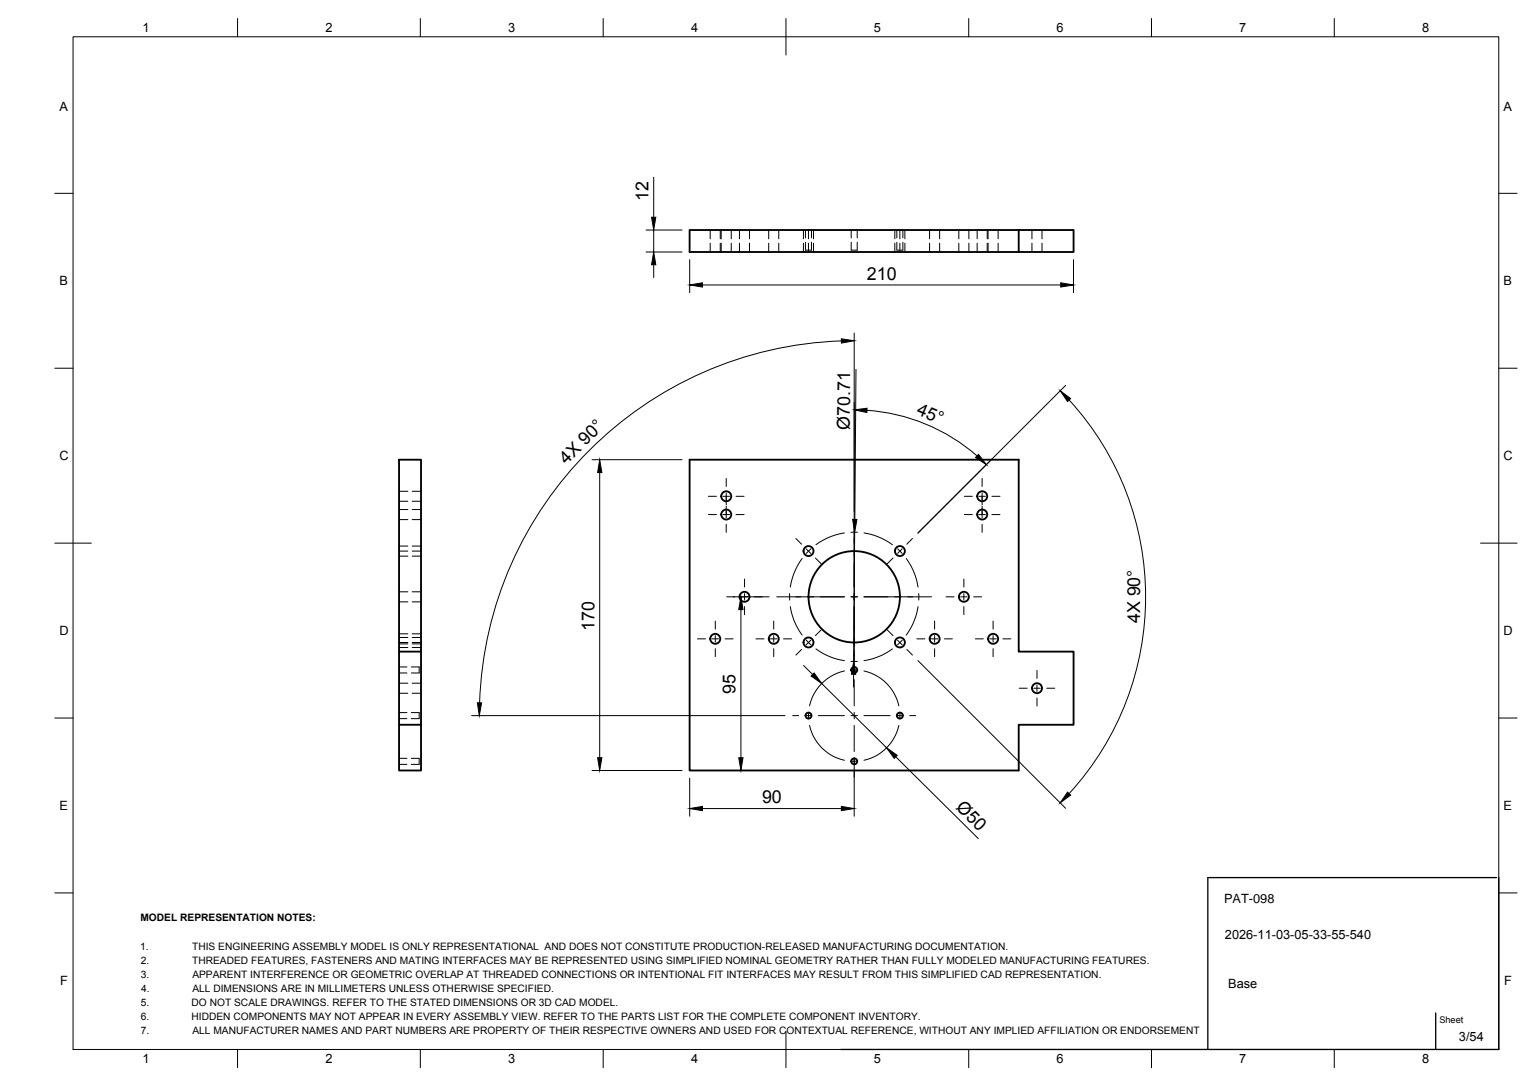
ISO-10303-21;
HEADER;
/* Generated by software containing ST-Developer
 * from STEP Tools, Inc. (www.steptools.com) 
 */

FILE_DESCRIPTION(
/* description */ ('Spring compression tester'),
/* implementation_level */ '2;1');

FILE_NAME(
/* name */ 'Base.step',
/* time_stamp */ '2026-10-28T03:24:11-07:00',
/* author */ (''),
/* organization */ (''),
/* preprocessor_version */ 'ST-DEVELOPER v20.2',
/* originating_system */ 'Autodesk Translation Framework v15.17.0.0',
/* authorisation */ '');

FILE_SCHEMA (('AUTOMOTIVE_DESIGN { 1 0 10303 214 3 1 1 }'));
ENDSEC;

DATA;
#10=MECHANICAL_DESIGN_GEOMETRIC_PRESENTATION_REPRESENTATION('',(#1104),#43521);
#984=SHAPE_REPRESENTATION_RELATIONSHIP('SRR','None',#43796,#1044);
#1044=ADVANCED_BREP_SHAPE_REPRESENTATION('',(#1179),#43456);
#1104=STYLED_ITEM('',(#44181),#1179);
#1179=MANIFOLD_SOLID_BREP('Body1',#18541);
#1247=FACE_BOUND('',#3250,.T.);
#1248=FACE_BOUND('',#3251,.T.);
#1249=FACE_BOUND('',#3252,.T.);
#1250=FACE_BOUND('',#3253,.T.);
#1251=FACE_BOUND('',#3254,.T.);
#1252=FACE_BOUND('',#3255,.T.);
#1253=FACE_BOUND('',#3256,.T.);
#1254=FACE_BOUND('',#3257,.T.);
#1255=FACE_BOUND('',#3258,.T.);
#1256=FACE_BOUND('',#3259,.T.);
#1257=FACE_BOUND('',#3260,.T.);
#1258=FACE_BOUND('',#3261,.T.);
#1259=FACE_BOUND('',#3262,.T.);
#1260=FACE_BOUND('',#3263,.T.);
#1261=FACE_BOUND('',#3264,.T.);
#1262=FACE_BOUND('',#3265,.T.);
#1263=FACE_BOUND('',#3266,.T.);
#1264=FACE_BOUND('',#3267,.T.);
#1265=FACE_BOUND('',#3268,.T.);
#1266=FACE_BOUND('',#3269,.T.);
#1267=FACE_BOUND('',#3271,.T.);
#1268=FACE_BOUND('',#3272,.T.);
#1269=FACE_BOUND('',#3273,.T.);
#1270=FACE_BOUND('',#3274,.T.);
#1271=FACE_BOUND('',#3275,.T.);
#1272=FACE_BOUND('',#3276,.T.);
#1273=FACE_BOUND('',#3277,.T.);
#1274=FACE_BOUND('',#3278,.T.);
#1275=FACE_BOUND('',#3279,.T.);
#1276=FACE_BOUND('',#3280,.T.);
#1277=FACE_BOUND('',#3281,.T.);
#1278=FACE_BOUND('',#3282,.T.);
#1279=FACE_BOUND('',#3283,.T.);
#1280=FACE_BOUND('',#3284,.T.);
#1281=FACE_BOUND('',#3285,.T.);
#1282=FACE_BOUND('',#3286,.T.);
#1589=PLANE('',#19290);
#1590=PLANE('',#19291);
#1591=PLANE('',#19292);
#1592=PLANE('',#19293);
#1593=PLANE('',#19294);
#1594=PLANE('',#19298);
#1595=PLANE('',#19302);
#1596=PLANE('',#19306);
#1597=PLANE('',#19310);
#1598=PLANE('',#19356);
#1599=PLANE('',#19357);
#1600=PLANE('',#19358);
#1601=PLANE('',#19359);
#1602=PLANE('',#19360);
#2170=FACE_OUTER_BOUND('',#3217,.T.);
#2171=FACE_OUTER_BOUND('',#3218,.T.);
#2172=FACE_OUTER_BOUND('',#3219,.T.);
#2173=FACE_OUTER_BOUND('',#3220,.T.);
#2174=FACE_OUTER_BOUND('',#3221,.T.);
#2175=FACE_OUTER_BOUND('',#3222,.T.);
#2176=FACE_OUTER_BOUND('',#3223,.T.);
#2177=FACE_OUTER_BOUND('',#3224,.T.);
#2178=FACE_OUTER_BOUND('',#3225,.T.);
#2179=FACE_OUTER_BOUND('',#3226,.T.);
#2180=FACE_OUTER_BOUND('',#3227,.T.);
#2181=FACE_OUTER_BOUND('',#3228,.T.);
#2182=FACE_OUTER_BOUND('',#3229,.T.);
#2183=FACE_OUTER_BOUND('',#3230,.T.);
#2184=FACE_OUTER_BOUND('',#3231,.T.);
#2185=FACE_OUTER_BOUND('',#3232,.T.);
#2186=FACE_OUTER_BOUND('',#3233,.T.);
#2187=FACE_OUTER_BOUND('',#3234,.T.);
#2188=FACE_OUTER_BOUND('',#3235,.T.);
#2189=FACE_OUTER_BOUND('',#3236,.T.);
#2190=FACE_OUTER_BOUND('',#3237,.T.);
#2191=FACE_OUTER_BOUND('',#3238,.T.);
#2192=FACE_OUTER_BOUND('',#3239,.T.);
#2193=FACE_OUTER_BOUND('',#3240,.T.);
#2194=FACE_OUTER_BOUND('',#3241,.T.);
#2195=FACE_OUTER_BOUND('',#3242,.T.);
#2196=FACE_OUTER_BOUND('',#3243,.T.);
#2197=FACE_OUTER_BOUND('',#3244,.T.);
#2198=FACE_OUTER_BOUND('',#3245,.T.);
#2199=FACE_OUTER_BOUND('',#3246,.T.);
#2200=FACE_OUTER_BOUND('',#3247,.T.);
#2201=FACE_OUTER_BOUND('',#3248,.T.);
#2202=FACE_OUTER_BOUND('',#3249,.T.);
#2203=FACE_OUTER_BOUND('',#3270,.T.);
#3217=EDGE_LOOP('',(#12217,#12218,#12219,#12220));
#3218=EDGE_LOOP('',(#12221,#12222,#12223,#12224));
#3219=EDGE_LOOP('',(#12225,#12226,#12227,#12228));
#3220=EDGE_LOOP('',(#12229,#12230,#12231,#12232));
#3221=EDGE_LOOP('',(#12233,#12234,#12235,#12236));
#3222=EDGE_LOOP('',(#12237,#12238,#12239,#12240));
#3223=EDGE_LOOP('',(#12241,#12242,#12243,#12244));
#3224=EDGE_LOOP('',(#12245));
#3225=EDGE_LOOP('',(#12246,#12247,#12248,#12249));
#3226=EDGE_LOOP('',(#12250));
#3227=EDGE_LOOP('',(#12251,#12252,#12253,#12254));
#3228=EDGE_LOOP('',(#12255));
#3229=EDGE_LOOP('',(#12256,#12257,#12258,#12259));
#3230=EDGE_LOOP('',(#12260));
#3231=EDGE_LOOP('',(#12261,#12262,#12263,#12264));
#3232=EDGE_LOOP('',(#12265,#12266,#12267,#12268));
#3233=EDGE_LOOP('',(#12269,#12270,#12271,#12272));
#3234=EDGE_LOOP('',(#12273,#12274,#12275,#12276));
#3235=EDGE_LOOP('',(#12277,#12278,#12279,#12280));
#3236=EDGE_LOOP('',(#12281,#12282,#12283,#12284));
#3237=EDGE_LOOP('',(#12285,#12286,#12287,#12288));
#3238=EDGE_LOOP('',(#12289,#12290,#12291,#12292));
#3239=EDGE_LOOP('',(#12293,#12294,#12295,#12296));
#3240=EDGE_LOOP('',(#12297,#12298,#12299,#12300));
#3241=EDGE_LOOP('',(#12301,#12302,#12303,#12304));
#3242=EDGE_LOOP('',(#12305,#12306,#12307,#12308));
#3243=EDGE_LOOP('',(#12309,#12310,#12311,#12312));
#3244=EDGE_LOOP('',(#12313,#12314,#12315,#12316));
#3245=EDGE_LOOP('',(#12317,#12318,#12319,#12320));
#3246=EDGE_LOOP('',(#12321,#12322,#12323,#12324));
#3247=EDGE_LOOP('',(#12325,#12326,#12327,#12328));
#3248=EDGE_LOOP('',(#12329,#12330,#12331,#12332));
#3249=EDGE_LOOP('',(#12333,#12334,#12335,#12336,#12337,#12338,#12339,#12340));
#3250=EDGE_LOOP('',(#12341));
#3251=EDGE_LOOP('',(#12342));
#3252=EDGE_LOOP('',(#12343));
#3253=EDGE_LOOP('',(#12344));
#3254=EDGE_LOOP('',(#12345));
#3255=EDGE_LOOP('',(#12346));
#3256=EDGE_LOOP('',(#12347));
#3257=EDGE_LOOP('',(#12348));
#3258=EDGE_LOOP('',(#12349));
#3259=EDGE_LOOP('',(#12350));
#3260=EDGE_LOOP('',(#12351));
#3261=EDGE_LOOP('',(#12352));
#3262=EDGE_LOOP('',(#12353));
#3263=EDGE_LOOP('',(#12354));
#3264=EDGE_LOOP('',(#12355));
#3265=EDGE_LOOP('',(#12356));
#3266=EDGE_LOOP('',(#12357));
#3267=EDGE_LOOP('',(#12358));
#3268=EDGE_LOOP('',(#12359));
#3269=EDGE_LOOP('',(#12360));
#3270=EDGE_LOOP('',(#12361,#12362,#12363,#12364,#12365,#12366,#12367,#12368));
#3271=EDGE_LOOP('',(#12369));
#3272=EDGE_LOOP('',(#12370));
#3273=EDGE_LOOP('',(#12371));
#3274=EDGE_LOOP('',(#12372));
#3275=EDGE_LOOP('',(#12373));
#3276=EDGE_LOOP('',(#12374));
#3277=EDGE_LOOP('',(#12375));
#3278=EDGE_LOOP('',(#12376));
#3279=EDGE_LOOP('',(#12377));
#3280=EDGE_LOOP('',(#12378));
#3281=EDGE_LOOP('',(#12379));
#3282=EDGE_LOOP('',(#12380));
#3283=EDGE_LOOP('',(#12381));
#3284=EDGE_LOOP('',(#12382));
#3285=EDGE_LOOP('',(#12383));
#3286=EDGE_LOOP('',(#12384));
#4606=LINE('',#26459,#6038);
#4607=LINE('',#26464,#6039);
#4608=LINE('',#26466,#6040);
#4609=LINE('',#26468,#6041);
#4610=LINE('',#26469,#6042);
#4611=LINE('',#26473,#6043);
#4612=LINE('',#26474,#6044);
#4613=LINE('',#26475,#6045);
#4614=LINE('',#26479,#6046);
#4615=LINE('',#26480,#6047);
#4616=LINE('',#26481,#6048);
#4617=LINE('',#26484,#6049);
#4618=LINE('',#26486,#6050);
#4619=LINE('',#26487,#6051);
#4620=LINE('',#26490,#6052);
#4621=LINE('',#26492,#6053);
#4622=LINE('',#26493,#6054);
#4623=LINE('',#26498,#6055);
#4624=LINE('',#26505,#6056);
#4625=LINE('',#26512,#6057);
#4626=LINE('',#26519,#6058);
#4627=LINE('',#26526,#6059);
#4628=LINE('',#26532,#6060);
#4629=LINE('',#26538,#6061);
#4630=LINE('',#26544,#6062);
#4631=LINE('',#26550,#6063);
#4632=LINE('',#26556,#6064);
#4633=LINE('',#26562,#6065);
#4634=LINE('',#26568,#6066);
#4635=LINE('',#26574,#6067);
#4636=LINE('',#26580,#6068);
#4637=LINE('',#26586,#6069);
#4638=LINE('',#26592,#6070);
#4639=LINE('',#26598,#6071);
#4640=LINE('',#26604,#6072);
#4641=LINE('',#26610,#6073);
#4642=LINE('',#26614,#6074);
#4643=LINE('',#26616,#6075);
#4644=LINE('',#26617,#6076);
#4645=LINE('',#26620,#6077);
#4646=LINE('',#26622,#6078);
#4647=LINE('',#26623,#6079);
#4648=LINE('',#26625,#6080);
#4649=LINE('',#26626,#6081);
#6038=VECTOR('',#21206,0.275);
#6039=VECTOR('',#21211,1.);
#6040=VECTOR('',#21212,1.);
#6041=VECTOR('',#21213,1.);
#6042=VECTOR('',#21214,1.);
#6043=VECTOR('',#21217,1.);
#6044=VECTOR('',#21218,1.);
#6045=VECTOR('',#21219,1.);
#6046=VECTOR('',#21222,1.);
#6047=VECTOR('',#21223,1.);
#6048=VECTOR('',#21224,1.);
#6049=VECTOR('',#21227,1.);
#6050=VECTOR('',#21228,1.);
#6051=VECTOR('',#21229,1.);
#6052=VECTOR('',#21232,1.);
#6053=VECTOR('',#21233,1.);
#6054=VECTOR('',#21234,1.);
#6055=VECTOR('',#21239,0.165);
#6056=VECTOR('',#21248,0.165);
#6057=VECTOR('',#21257,0.165);
#6058=VECTOR('',#21266,0.165);
#6059=VECTOR('',#21275,0.275);
#6060=VECTOR('',#21282,0.275);
#6061=VECTOR('',#21289,0.275);
#6062=VECTOR('',#21296,0.275);
#6063=VECTOR('',#21303,0.275);
#6064=VECTOR('',#21310,0.275);
#6065=VECTOR('',#21317,2.5);
#6066=VECTOR('',#21324,0.275);
#6067=VECTOR('',#21331,0.275);
#6068=VECTOR('',#21338,0.275);
#6069=VECTOR('',#21345,0.275);
#6070=VECTOR('',#21352,0.275);
#6071=VECTOR('',#21359,0.275);
#6072=VECTOR('',#21366,0.275);
#6073=VECTOR('',#21373,0.275);
#6074=VECTOR('',#21378,1.);
#6075=VECTOR('',#21379,1.);
#6076=VECTOR('',#21380,1.);
#6077=VECTOR('',#21383,1.);
#6078=VECTOR('',#21384,1.);
#6079=VECTOR('',#21385,1.);
#6080=VECTOR('',#21388,1.);
#6081=VECTOR('',#21389,1.);
#7470=CIRCLE('',#19288,0.275);
#7471=CIRCLE('',#19289,0.275);
#7472=CIRCLE('',#19296,0.165);
#7473=CIRCLE('',#19297,0.165);
#7474=CIRCLE('',#19300,0.165);
#7475=CIRCLE('',#19301,0.165);
#7476=CIRCLE('',#19304,0.165);
#7477=CIRCLE('',#19305,0.165);
#7478=CIRCLE('',#19308,0.165);
#7479=CIRCLE('',#19309,0.165);
#7480=CIRCLE('',#19312,0.275);
#7481=CIRCLE('',#19313,0.275);
#7482=CIRCLE('',#19315,0.275);
#7483=CIRCLE('',#19316,0.275);
#7484=CIRCLE('',#19318,0.275);
#7485=CIRCLE('',#19319,0.275);
#7486=CIRCLE('',#19321,0.275);
#7487=CIRCLE('',#19322,0.275);
#7488=CIRCLE('',#19324,0.275);
#7489=CIRCLE('',#19325,0.275);
#7490=CIRCLE('',#19327,0.275);
#7491=CIRCLE('',#19328,0.275);
#7492=CIRCLE('',#19330,2.5);
#7493=CIRCLE('',#19331,2.5);
#7494=CIRCLE('',#19333,0.275);
#7495=CIRCLE('',#19334,0.275);
#7496=CIRCLE('',#19336,0.275);
#7497=CIRCLE('',#19337,0.275);
#7498=CIRCLE('',#19339,0.275);
#7499=CIRCLE('',#19340,0.275);
#7500=CIRCLE('',#19342,0.275);
#7501=CIRCLE('',#19343,0.275);
#7502=CIRCLE('',#19345,0.275);
#7503=CIRCLE('',#19346,0.275);
#7504=CIRCLE('',#19348,0.275);
#7505=CIRCLE('',#19349,0.275);
#7506=CIRCLE('',#19351,0.275);
#7507=CIRCLE('',#19352,0.275);
#7508=CIRCLE('',#19354,0.275);
#7509=CIRCLE('',#19355,0.275);
#8136=VERTEX_POINT('',#26456);
#8137=VERTEX_POINT('',#26458);
#8138=VERTEX_POINT('',#26462);
#8139=VERTEX_POINT('',#26463);
#8140=VERTEX_POINT('',#26465);
#8141=VERTEX_POINT('',#26467);
#8142=VERTEX_POINT('',#26471);
#8143=VERTEX_POINT('',#26472);
#8144=VERTEX_POINT('',#26477);
#8145=VERTEX_POINT('',#26478);
#8146=VERTEX_POINT('',#26483);
#8147=VERTEX_POINT('',#26485);
#8148=VERTEX_POINT('',#26489);
#8149=VERTEX_POINT('',#26491);
#8150=VERTEX_POINT('',#26495);
#8151=VERTEX_POINT('',#26497);
#8152=VERTEX_POINT('',#26502);
#8153=VERTEX_POINT('',#26504);
#8154=VERTEX_POINT('',#26509);
#8155=VERTEX_POINT('',#26511);
#8156=VERTEX_POINT('',#26516);
#8157=VERTEX_POINT('',#26518);
#8158=VERTEX_POINT('',#26523);
#8159=VERTEX_POINT('',#26525);
#8160=VERTEX_POINT('',#26529);
#8161=VERTEX_POINT('',#26531);
#8162=VERTEX_POINT('',#26535);
#8163=VERTEX_POINT('',#26537);
#8164=VERTEX_POINT('',#26541);
#8165=VERTEX_POINT('',#26543);
#8166=VERTEX_POINT('',#26547);
#8167=VERTEX_POINT('',#26549);
#8168=VERTEX_POINT('',#26553);
#8169=VERTEX_POINT('',#26555);
#8170=VERTEX_POINT('',#26559);
#8171=VERTEX_POINT('',#26561);
#8172=VERTEX_POINT('',#26565);
#8173=VERTEX_POINT('',#26567);
#8174=VERTEX_POINT('',#26571);
#8175=VERTEX_POINT('',#26573);
#8176=VERTEX_POINT('',#26577);
#8177=VERTEX_POINT('',#26579);
#8178=VERTEX_POINT('',#26583);
#8179=VERTEX_POINT('',#26585);
#8180=VERTEX_POINT('',#26589);
#8181=VERTEX_POINT('',#26591);
#8182=VERTEX_POINT('',#26595);
#8183=VERTEX_POINT('',#26597);
#8184=VERTEX_POINT('',#26601);
#8185=VERTEX_POINT('',#26603);
#8186=VERTEX_POINT('',#26607);
#8187=VERTEX_POINT('',#26609);
#8188=VERTEX_POINT('',#26613);
#8189=VERTEX_POINT('',#26615);
#8190=VERTEX_POINT('',#26619);
#8191=VERTEX_POINT('',#26621);
#9773=EDGE_CURVE('',#8136,#8136,#7470,.T.);
#9774=EDGE_CURVE('',#8136,#8137,#4606,.T.);
#9775=EDGE_CURVE('',#8137,#8137,#7471,.T.);
#9776=EDGE_CURVE('',#8138,#8139,#4607,.T.);
#9777=EDGE_CURVE('',#8138,#8140,#4608,.T.);
#9778=EDGE_CURVE('',#8140,#8141,#4609,.T.);
#9779=EDGE_CURVE('',#8141,#8139,#4610,.T.);
#9780=EDGE_CURVE('',#8142,#8143,#4611,.T.);
#9781=EDGE_CURVE('',#8142,#8141,#4612,.T.);
#9782=EDGE_CURVE('',#8143,#8140,#4613,.T.);
#9783=EDGE_CURVE('',#8144,#8145,#4614,.T.);
#9784=EDGE_CURVE('',#8144,#8142,#4615,.T.);
#9785=EDGE_CURVE('',#8143,#8145,#4616,.T.);
#9786=EDGE_CURVE('',#8139,#8146,#4617,.T.);
#9787=EDGE_CURVE('',#8146,#8147,#4618,.T.);
#9788=EDGE_CURVE('',#8138,#8147,#4619,.T.);
#9789=EDGE_CURVE('',#8148,#8145,#4620,.T.);
#9790=EDGE_CURVE('',#8149,#8148,#4621,.T.);
#9791=EDGE_CURVE('',#8149,#8144,#4622,.T.);
#9792=EDGE_CURVE('',#8150,#8150,#7472,.T.);
#9793=EDGE_CURVE('',#8150,#8151,#4623,.T.);
#9794=EDGE_CURVE('',#8151,#8151,#7473,.T.);
#9795=EDGE_CURVE('',#8152,#8152,#7474,.T.);
#9796=EDGE_CURVE('',#8152,#8153,#4624,.T.);
#9797=EDGE_CURVE('',#8153,#8153,#7475,.T.);
#9798=EDGE_CURVE('',#8154,#8154,#7476,.T.);
#9799=EDGE_CURVE('',#8154,#8155,#4625,.T.);
#9800=EDGE_CURVE('',#8155,#8155,#7477,.T.);
#9801=EDGE_CURVE('',#8156,#8156,#7478,.T.);
#9802=EDGE_CURVE('',#8156,#8157,#4626,.T.);
#9803=EDGE_CURVE('',#8157,#8157,#7479,.T.);
#9804=EDGE_CURVE('',#8158,#8158,#7480,.T.);
#9805=EDGE_CURVE('',#8158,#8159,#4627,.T.);
#9806=EDGE_CURVE('',#8159,#8159,#7481,.T.);
#9807=EDGE_CURVE('',#8160,#8160,#7482,.T.);
#9808=EDGE_CURVE('',#8160,#8161,#4628,.T.);
#9809=EDGE_CURVE('',#8161,#8161,#7483,.T.);
#9810=EDGE_CURVE('',#8162,#8162,#7484,.T.);
#9811=EDGE_CURVE('',#8162,#8163,#4629,.T.);
#9812=EDGE_CURVE('',#8163,#8163,#7485,.T.);
#9813=EDGE_CURVE('',#8164,#8164,#7486,.T.);
#9814=EDGE_CURVE('',#8164,#8165,#4630,.T.);
#9815=EDGE_CURVE('',#8165,#8165,#7487,.T.);
#9816=EDGE_CURVE('',#8166,#8166,#7488,.T.);
#9817=EDGE_CURVE('',#8166,#8167,#4631,.T.);
#9818=EDGE_CURVE('',#8167,#8167,#7489,.T.);
#9819=EDGE_CURVE('',#8168,#8168,#7490,.T.);
#9820=EDGE_CURVE('',#8168,#8169,#4632,.T.);
#9821=EDGE_CURVE('',#8169,#8169,#7491,.T.);
#9822=EDGE_CURVE('',#8170,#8170,#7492,.T.);
#9823=EDGE_CURVE('',#8170,#8171,#4633,.T.);
#9824=EDGE_CURVE('',#8171,#8171,#7493,.T.);
#9825=EDGE_CURVE('',#8172,#8172,#7494,.T.);
#9826=EDGE_CURVE('',#8172,#8173,#4634,.T.);
#9827=EDGE_CURVE('',#8173,#8173,#7495,.T.);
#9828=EDGE_CURVE('',#8174,#8174,#7496,.T.);
#9829=EDGE_CURVE('',#8174,#8175,#4635,.T.);
#9830=EDGE_CURVE('',#8175,#8175,#7497,.T.);
#9831=EDGE_CURVE('',#8176,#8176,#7498,.T.);
#9832=EDGE_CURVE('',#8176,#8177,#4636,.T.);
#9833=EDGE_CURVE('',#8177,#8177,#7499,.T.);
#9834=EDGE_CURVE('',#8178,#8178,#7500,.T.);
#9835=EDGE_CURVE('',#8178,#8179,#4637,.T.);
#9836=EDGE_CURVE('',#8179,#8179,#7501,.T.);
#9837=EDGE_CURVE('',#8180,#8180,#7502,.T.);
#9838=EDGE_CURVE('',#8180,#8181,#4638,.T.);
#9839=EDGE_CURVE('',#8181,#8181,#7503,.T.);
#9840=EDGE_CURVE('',#8182,#8182,#7504,.T.);
#9841=EDGE_CURVE('',#8182,#8183,#4639,.T.);
#9842=EDGE_CURVE('',#8183,#8183,#7505,.T.);
#9843=EDGE_CURVE('',#8184,#8184,#7506,.T.);
#9844=EDGE_CURVE('',#8184,#8185,#4640,.T.);
#9845=EDGE_CURVE('',#8185,#8185,#7507,.T.);
#9846=EDGE_CURVE('',#8186,#8186,#7508,.T.);
#9847=EDGE_CURVE('',#8186,#8187,#4641,.T.);
#9848=EDGE_CURVE('',#8187,#8187,#7509,.T.);
#9849=EDGE_CURVE('',#8146,#8188,#4642,.T.);
#9850=EDGE_CURVE('',#8188,#8189,#4643,.T.);
#9851=EDGE_CURVE('',#8147,#8189,#4644,.T.);
#9852=EDGE_CURVE('',#8190,#8149,#4645,.T.);
#9853=EDGE_CURVE('',#8191,#8148,#4646,.T.);
#9854=EDGE_CURVE('',#8190,#8191,#4647,.T.);
#9855=EDGE_CURVE('',#8188,#8190,#4648,.T.);
#9856=EDGE_CURVE('',#8189,#8191,#4649,.T.);
#12217=ORIENTED_EDGE('',*,*,#9773,.F.);
#12218=ORIENTED_EDGE('',*,*,#9774,.T.);
#12219=ORIENTED_EDGE('',*,*,#9775,.F.);
#12220=ORIENTED_EDGE('',*,*,#9774,.F.);
#12221=ORIENTED_EDGE('',*,*,#9776,.F.);
#12222=ORIENTED_EDGE('',*,*,#9777,.T.);
#12223=ORIENTED_EDGE('',*,*,#9778,.T.);
#12224=ORIENTED_EDGE('',*,*,#9779,.T.);
#12225=ORIENTED_EDGE('',*,*,#9780,.F.);
#12226=ORIENTED_EDGE('',*,*,#9781,.T.);
#12227=ORIENTED_EDGE('',*,*,#9778,.F.);
#12228=ORIENTED_EDGE('',*,*,#9782,.F.);
#12229=ORIENTED_EDGE('',*,*,#9783,.F.);
#12230=ORIENTED_EDGE('',*,*,#9784,.T.);
#12231=ORIENTED_EDGE('',*,*,#9780,.T.);
#12232=ORIENTED_EDGE('',*,*,#9785,.T.);
#12233=ORIENTED_EDGE('',*,*,#9776,.T.);
#12234=ORIENTED_EDGE('',*,*,#9786,.T.);
#12235=ORIENTED_EDGE('',*,*,#9787,.T.);
#12236=ORIENTED_EDGE('',*,*,#9788,.F.);
#12237=ORIENTED_EDGE('',*,*,#9783,.T.);
#12238=ORIENTED_EDGE('',*,*,#9789,.F.);
#12239=ORIENTED_EDGE('',*,*,#9790,.F.);
#12240=ORIENTED_EDGE('',*,*,#9791,.T.);
#12241=ORIENTED_EDGE('',*,*,#9792,.F.);
#12242=ORIENTED_EDGE('',*,*,#9793,.T.);
#12243=ORIENTED_EDGE('',*,*,#9794,.F.);
#12244=ORIENTED_EDGE('',*,*,#9793,.F.);
#12245=ORIENTED_EDGE('',*,*,#9792,.T.);
#12246=ORIENTED_EDGE('',*,*,#9795,.F.);
#12247=ORIENTED_EDGE('',*,*,#9796,.T.);
#12248=ORIENTED_EDGE('',*,*,#9797,.F.);
#12249=ORIENTED_EDGE('',*,*,#9796,.F.);
#12250=ORIENTED_EDGE('',*,*,#9795,.T.);
#12251=ORIENTED_EDGE('',*,*,#9798,.F.);
#12252=ORIENTED_EDGE('',*,*,#9799,.T.);
#12253=ORIENTED_EDGE('',*,*,#9800,.F.);
#12254=ORIENTED_EDGE('',*,*,#9799,.F.);
#12255=ORIENTED_EDGE('',*,*,#9798,.T.);
#12256=ORIENTED_EDGE('',*,*,#9801,.F.);
#12257=ORIENTED_EDGE('',*,*,#9802,.T.);
#12258=ORIENTED_EDGE('',*,*,#9803,.F.);
#12259=ORIENTED_EDGE('',*,*,#9802,.F.);
#12260=ORIENTED_EDGE('',*,*,#9801,.T.);
#12261=ORIENTED_EDGE('',*,*,#9804,.F.);
#12262=ORIENTED_EDGE('',*,*,#9805,.T.);
#12263=ORIENTED_EDGE('',*,*,#9806,.F.);
#12264=ORIENTED_EDGE('',*,*,#9805,.F.);
#12265=ORIENTED_EDGE('',*,*,#9807,.F.);
#12266=ORIENTED_EDGE('',*,*,#9808,.T.);
#12267=ORIENTED_EDGE('',*,*,#9809,.F.);
#12268=ORIENTED_EDGE('',*,*,#9808,.F.);
#12269=ORIENTED_EDGE('',*,*,#9810,.F.);
#12270=ORIENTED_EDGE('',*,*,#9811,.T.);
#12271=ORIENTED_EDGE('',*,*,#9812,.F.);
#12272=ORIENTED_EDGE('',*,*,#9811,.F.);
#12273=ORIENTED_EDGE('',*,*,#9813,.F.);
#12274=ORIENTED_EDGE('',*,*,#9814,.T.);
#12275=ORIENTED_EDGE('',*,*,#9815,.F.);
#12276=ORIENTED_EDGE('',*,*,#9814,.F.);
#12277=ORIENTED_EDGE('',*,*,#9816,.F.);
#12278=ORIENTED_EDGE('',*,*,#9817,.T.);
#12279=ORIENTED_EDGE('',*,*,#9818,.F.);
#12280=ORIENTED_EDGE('',*,*,#9817,.F.);
#12281=ORIENTED_EDGE('',*,*,#9819,.F.);
#12282=ORIENTED_EDGE('',*,*,#9820,.T.);
#12283=ORIENTED_EDGE('',*,*,#9821,.F.);
#12284=ORIENTED_EDGE('',*,*,#9820,.F.);
#12285=ORIENTED_EDGE('',*,*,#9822,.F.);
#12286=ORIENTED_EDGE('',*,*,#9823,.T.);
#12287=ORIENTED_EDGE('',*,*,#9824,.F.);
#12288=ORIENTED_EDGE('',*,*,#9823,.F.);
#12289=ORIENTED_EDGE('',*,*,#9825,.F.);
#12290=ORIENTED_EDGE('',*,*,#9826,.T.);
#12291=ORIENTED_EDGE('',*,*,#9827,.F.);
#12292=ORIENTED_EDGE('',*,*,#9826,.F.);
#12293=ORIENTED_EDGE('',*,*,#9828,.F.);
#12294=ORIENTED_EDGE('',*,*,#9829,.T.);
#12295=ORIENTED_EDGE('',*,*,#9830,.F.);
#12296=ORIENTED_EDGE('',*,*,#9829,.F.);
#12297=ORIENTED_EDGE('',*,*,#9831,.F.);
#12298=ORIENTED_EDGE('',*,*,#9832,.T.);
#12299=ORIENTED_EDGE('',*,*,#9833,.F.);
#12300=ORIENTED_EDGE('',*,*,#9832,.F.);
#12301=ORIENTED_EDGE('',*,*,#9834,.F.);
#12302=ORIENTED_EDGE('',*,*,#9835,.T.);
#12303=ORIENTED_EDGE('',*,*,#9836,.F.);
#12304=ORIENTED_EDGE('',*,*,#9835,.F.);
#12305=ORIENTED_EDGE('',*,*,#9837,.F.);
#12306=ORIENTED_EDGE('',*,*,#9838,.T.);
#12307=ORIENTED_EDGE('',*,*,#9839,.F.);
#12308=ORIENTED_EDGE('',*,*,#9838,.F.);
#12309=ORIENTED_EDGE('',*,*,#9840,.F.);
#12310=ORIENTED_EDGE('',*,*,#9841,.T.);
#12311=ORIENTED_EDGE('',*,*,#9842,.F.);
#12312=ORIENTED_EDGE('',*,*,#9841,.F.);
#12313=ORIENTED_EDGE('',*,*,#9843,.F.);
#12314=ORIENTED_EDGE('',*,*,#9844,.T.);
#12315=ORIENTED_EDGE('',*,*,#9845,.F.);
#12316=ORIENTED_EDGE('',*,*,#9844,.F.);
#12317=ORIENTED_EDGE('',*,*,#9846,.F.);
#12318=ORIENTED_EDGE('',*,*,#9847,.T.);
#12319=ORIENTED_EDGE('',*,*,#9848,.F.);
#12320=ORIENTED_EDGE('',*,*,#9847,.F.);
#12321=ORIENTED_EDGE('',*,*,#9849,.T.);
#12322=ORIENTED_EDGE('',*,*,#9850,.T.);
#12323=ORIENTED_EDGE('',*,*,#9851,.F.);
#12324=ORIENTED_EDGE('',*,*,#9787,.F.);
#12325=ORIENTED_EDGE('',*,*,#9852,.T.);
#12326=ORIENTED_EDGE('',*,*,#9790,.T.);
#12327=ORIENTED_EDGE('',*,*,#9853,.F.);
#12328=ORIENTED_EDGE('',*,*,#9854,.F.);
#12329=ORIENTED_EDGE('',*,*,#9855,.T.);
#12330=ORIENTED_EDGE('',*,*,#9854,.T.);
#12331=ORIENTED_EDGE('',*,*,#9856,.F.);
#12332=ORIENTED_EDGE('',*,*,#9850,.F.);
#12333=ORIENTED_EDGE('',*,*,#9788,.T.);
#12334=ORIENTED_EDGE('',*,*,#9851,.T.);
#12335=ORIENTED_EDGE('',*,*,#9856,.T.);
#12336=ORIENTED_EDGE('',*,*,#9853,.T.);
#12337=ORIENTED_EDGE('',*,*,#9789,.T.);
#12338=ORIENTED_EDGE('',*,*,#9785,.F.);
#12339=ORIENTED_EDGE('',*,*,#9782,.T.);
#12340=ORIENTED_EDGE('',*,*,#9777,.F.);
#12341=ORIENTED_EDGE('',*,*,#9806,.T.);
#12342=ORIENTED_EDGE('',*,*,#9812,.T.);
#12343=ORIENTED_EDGE('',*,*,#9815,.T.);
#12344=ORIENTED_EDGE('',*,*,#9818,.T.);
#12345=ORIENTED_EDGE('',*,*,#9821,.T.);
#12346=ORIENTED_EDGE('',*,*,#9827,.T.);
#12347=ORIENTED_EDGE('',*,*,#9830,.T.);
#12348=ORIENTED_EDGE('',*,*,#9833,.T.);
#12349=ORIENTED_EDGE('',*,*,#9836,.T.);
#12350=ORIENTED_EDGE('',*,*,#9839,.T.);
#12351=ORIENTED_EDGE('',*,*,#9842,.T.);
#12352=ORIENTED_EDGE('',*,*,#9845,.T.);
#12353=ORIENTED_EDGE('',*,*,#9848,.T.);
#12354=ORIENTED_EDGE('',*,*,#9824,.T.);
#12355=ORIENTED_EDGE('',*,*,#9809,.T.);
#12356=ORIENTED_EDGE('',*,*,#9803,.T.);
#12357=ORIENTED_EDGE('',*,*,#9800,.T.);
#12358=ORIENTED_EDGE('',*,*,#9797,.T.);
#12359=ORIENTED_EDGE('',*,*,#9794,.T.);
#12360=ORIENTED_EDGE('',*,*,#9775,.T.);
#12361=ORIENTED_EDGE('',*,*,#9791,.F.);
#12362=ORIENTED_EDGE('',*,*,#9852,.F.);
#12363=ORIENTED_EDGE('',*,*,#9855,.F.);
#12364=ORIENTED_EDGE('',*,*,#9849,.F.);
#12365=ORIENTED_EDGE('',*,*,#9786,.F.);
#12366=ORIENTED_EDGE('',*,*,#9779,.F.);
#12367=ORIENTED_EDGE('',*,*,#9781,.F.);
#12368=ORIENTED_EDGE('',*,*,#9784,.F.);
#12369=ORIENTED_EDGE('',*,*,#9807,.T.);
#12370=ORIENTED_EDGE('',*,*,#9822,.T.);
#12371=ORIENTED_EDGE('',*,*,#9846,.T.);
#12372=ORIENTED_EDGE('',*,*,#9843,.T.);
#12373=ORIENTED_EDGE('',*,*,#9840,.T.);
#12374=ORIENTED_EDGE('',*,*,#9837,.T.);
#12375=ORIENTED_EDGE('',*,*,#9834,.T.);
#12376=ORIENTED_EDGE('',*,*,#9831,.T.);
#12377=ORIENTED_EDGE('',*,*,#9828,.T.);
#12378=ORIENTED_EDGE('',*,*,#9825,.T.);
#12379=ORIENTED_EDGE('',*,*,#9819,.T.);
#12380=ORIENTED_EDGE('',*,*,#9816,.T.);
#12381=ORIENTED_EDGE('',*,*,#9813,.T.);
#12382=ORIENTED_EDGE('',*,*,#9810,.T.);
#12383=ORIENTED_EDGE('',*,*,#9804,.T.);
#12384=ORIENTED_EDGE('',*,*,#9773,.T.);
#17105=CYLINDRICAL_SURFACE('',#19287,0.275);
#17106=CYLINDRICAL_SURFACE('',#19295,0.165);
#17107=CYLINDRICAL_SURFACE('',#19299,0.165);
#17108=CYLINDRICAL_SURFACE('',#19303,0.165);
#17109=CYLINDRICAL_SURFACE('',#19307,0.165);
#17110=CYLINDRICAL_SURFACE('',#19311,0.275);
#17111=CYLINDRICAL_SURFACE('',#19314,0.275);
#17112=CYLINDRICAL_SURFACE('',#19317,0.275);
#17113=CYLINDRICAL_SURFACE('',#19320,0.275);
#17114=CYLINDRICAL_SURFACE('',#19323,0.275);
#17115=CYLINDRICAL_SURFACE('',#19326,0.275);
#17116=CYLINDRICAL_SURFACE('',#19329,2.5);
#17117=CYLINDRICAL_SURFACE('',#19332,0.275);
#17118=CYLINDRICAL_SURFACE('',#19335,0.275);
#17119=CYLINDRICAL_SURFACE('',#19338,0.275);
#17120=CYLINDRICAL_SURFACE('',#19341,0.275);
#17121=CYLINDRICAL_SURFACE('',#19344,0.275);
#17122=CYLINDRICAL_SURFACE('',#19347,0.275);
#17123=CYLINDRICAL_SURFACE('',#19350,0.275);
#17124=CYLINDRICAL_SURFACE('',#19353,0.275);
#17494=ADVANCED_FACE('',(#2170),#17105,.F.);
#17495=ADVANCED_FACE('',(#2171),#1589,.T.);
#17496=ADVANCED_FACE('',(#2172),#1590,.T.);
#17497=ADVANCED_FACE('',(#2173),#1591,.F.);
#17498=ADVANCED_FACE('',(#2174),#1592,.T.);
#17499=ADVANCED_FACE('',(#2175),#1593,.T.);
#17500=ADVANCED_FACE('',(#2176),#17106,.F.);
#17501=ADVANCED_FACE('',(#2177),#1594,.T.);
#17502=ADVANCED_FACE('',(#2178),#17107,.F.);
#17503=ADVANCED_FACE('',(#2179),#1595,.T.);
#17504=ADVANCED_FACE('',(#2180),#17108,.F.);
#17505=ADVANCED_FACE('',(#2181),#1596,.T.);
#17506=ADVANCED_FACE('',(#2182),#17109,.F.);
#17507=ADVANCED_FACE('',(#2183),#1597,.T.);
#17508=ADVANCED_FACE('',(#2184),#17110,.F.);
#17509=ADVANCED_FACE('',(#2185),#17111,.F.);
#17510=ADVANCED_FACE('',(#2186),#17112,.F.);
#17511=ADVANCED_FACE('',(#2187),#17113,.F.);
#17512=ADVANCED_FACE('',(#2188),#17114,.F.);
#17513=ADVANCED_FACE('',(#2189),#17115,.F.);
#17514=ADVANCED_FACE('',(#2190),#17116,.F.);
#17515=ADVANCED_FACE('',(#2191),#17117,.F.);
#17516=ADVANCED_FACE('',(#2192),#17118,.F.);
#17517=ADVANCED_FACE('',(#2193),#17119,.F.);
#17518=ADVANCED_FACE('',(#2194),#17120,.F.);
#17519=ADVANCED_FACE('',(#2195),#17121,.F.);
#17520=ADVANCED_FACE('',(#2196),#17122,.F.);
#17521=ADVANCED_FACE('',(#2197),#17123,.F.);
#17522=ADVANCED_FACE('',(#2198),#17124,.F.);
#17523=ADVANCED_FACE('',(#2199),#1598,.T.);
#17524=ADVANCED_FACE('',(#2200),#1599,.T.);
#17525=ADVANCED_FACE('',(#2201),#1600,.T.);
#17526=ADVANCED_FACE('',(#2202,#1247,#1248,#1249,#1250,#1251,#1252,#1253,
#1254,#1255,#1256,#1257,#1258,#1259,#1260,#1261,#1262,#1263,#1264,#1265,
#1266),#1601,.T.);
#17527=ADVANCED_FACE('',(#2203,#1267,#1268,#1269,#1270,#1271,#1272,#1273,
#1274,#1275,#1276,#1277,#1278,#1279,#1280,#1281,#1282),#1602,.F.);
#18541=CLOSED_SHELL('',(#17494,#17495,#17496,#17497,#17498,#17499,#17500,
#17501,#17502,#17503,#17504,#17505,#17506,#17507,#17508,#17509,#17510,#17511,
#17512,#17513,#17514,#17515,#17516,#17517,#17518,#17519,#17520,#17521,#17522,
#17523,#17524,#17525,#17526,#17527));
#19286=AXIS2_PLACEMENT_3D('',#26454,#21200,#21201);
#19287=AXIS2_PLACEMENT_3D('',#26455,#21202,#21203);
#19288=AXIS2_PLACEMENT_3D('',#26457,#21204,#21205);
#19289=AXIS2_PLACEMENT_3D('',#26460,#21207,#21208);
#19290=AXIS2_PLACEMENT_3D('',#26461,#21209,#21210);
#19291=AXIS2_PLACEMENT_3D('',#26470,#21215,#21216);
#19292=AXIS2_PLACEMENT_3D('',#26476,#21220,#21221);
#19293=AXIS2_PLACEMENT_3D('',#26482,#21225,#21226);
#19294=AXIS2_PLACEMENT_3D('',#26488,#21230,#21231);
#19295=AXIS2_PLACEMENT_3D('',#26494,#21235,#21236);
#19296=AXIS2_PLACEMENT_3D('',#26496,#21237,#21238);
#19297=AXIS2_PLACEMENT_3D('',#26499,#21240,#21241);
#19298=AXIS2_PLACEMENT_3D('',#26500,#21242,#21243);
#19299=AXIS2_PLACEMENT_3D('',#26501,#21244,#21245);
#19300=AXIS2_PLACEMENT_3D('',#26503,#21246,#21247);
#19301=AXIS2_PLACEMENT_3D('',#26506,#21249,#21250);
#19302=AXIS2_PLACEMENT_3D('',#26507,#21251,#21252);
#19303=AXIS2_PLACEMENT_3D('',#26508,#21253,#21254);
#19304=AXIS2_PLACEMENT_3D('',#26510,#21255,#21256);
#19305=AXIS2_PLACEMENT_3D('',#26513,#21258,#21259);
#19306=AXIS2_PLACEMENT_3D('',#26514,#21260,#21261);
#19307=AXIS2_PLACEMENT_3D('',#26515,#21262,#21263);
#19308=AXIS2_PLACEMENT_3D('',#26517,#21264,#21265);
#19309=AXIS2_PLACEMENT_3D('',#26520,#21267,#21268);
#19310=AXIS2_PLACEMENT_3D('',#26521,#21269,#21270);
#19311=AXIS2_PLACEMENT_3D('',#26522,#21271,#21272);
#19312=AXIS2_PLACEMENT_3D('',#26524,#21273,#21274);
#19313=AXIS2_PLACEMENT_3D('',#26527,#21276,#21277);
#19314=AXIS2_PLACEMENT_3D('',#26528,#21278,#21279);
#19315=AXIS2_PLACEMENT_3D('',#26530,#21280,#21281);
#19316=AXIS2_PLACEMENT_3D('',#26533,#21283,#21284);
#19317=AXIS2_PLACEMENT_3D('',#26534,#21285,#21286);
#19318=AXIS2_PLACEMENT_3D('',#26536,#21287,#21288);
#19319=AXIS2_PLACEMENT_3D('',#26539,#21290,#21291);
#19320=AXIS2_PLACEMENT_3D('',#26540,#21292,#21293);
#19321=AXIS2_PLACEMENT_3D('',#26542,#21294,#21295);
#19322=AXIS2_PLACEMENT_3D('',#26545,#21297,#21298);
#19323=AXIS2_PLACEMENT_3D('',#26546,#21299,#21300);
#19324=AXIS2_PLACEMENT_3D('',#26548,#21301,#21302);
#19325=AXIS2_PLACEMENT_3D('',#26551,#21304,#21305);
#19326=AXIS2_PLACEMENT_3D('',#26552,#21306,#21307);
#19327=AXIS2_PLACEMENT_3D('',#26554,#21308,#21309);
#19328=AXIS2_PLACEMENT_3D('',#26557,#21311,#21312);
#19329=AXIS2_PLACEMENT_3D('',#26558,#21313,#21314);
#19330=AXIS2_PLACEMENT_3D('',#26560,#21315,#21316);
#19331=AXIS2_PLACEMENT_3D('',#26563,#21318,#21319);
#19332=AXIS2_PLACEMENT_3D('',#26564,#21320,#21321);
#19333=AXIS2_PLACEMENT_3D('',#26566,#21322,#21323);
#19334=AXIS2_PLACEMENT_3D('',#26569,#21325,#21326);
#19335=AXIS2_PLACEMENT_3D('',#26570,#21327,#21328);
#19336=AXIS2_PLACEMENT_3D('',#26572,#21329,#21330);
#19337=AXIS2_PLACEMENT_3D('',#26575,#21332,#21333);
#19338=AXIS2_PLACEMENT_3D('',#26576,#21334,#21335);
#19339=AXIS2_PLACEMENT_3D('',#26578,#21336,#21337);
#19340=AXIS2_PLACEMENT_3D('',#26581,#21339,#21340);
#19341=AXIS2_PLACEMENT_3D('',#26582,#21341,#21342);
#19342=AXIS2_PLACEMENT_3D('',#26584,#21343,#21344);
#19343=AXIS2_PLACEMENT_3D('',#26587,#21346,#21347);
#19344=AXIS2_PLACEMENT_3D('',#26588,#21348,#21349);
#19345=AXIS2_PLACEMENT_3D('',#26590,#21350,#21351);
#19346=AXIS2_PLACEMENT_3D('',#26593,#21353,#21354);
#19347=AXIS2_PLACEMENT_3D('',#26594,#21355,#21356);
#19348=AXIS2_PLACEMENT_3D('',#26596,#21357,#21358);
#19349=AXIS2_PLACEMENT_3D('',#26599,#21360,#21361);
#19350=AXIS2_PLACEMENT_3D('',#26600,#21362,#21363);
#19351=AXIS2_PLACEMENT_3D('',#26602,#21364,#21365);
#19352=AXIS2_PLACEMENT_3D('',#26605,#21367,#21368);
#19353=AXIS2_PLACEMENT_3D('',#26606,#21369,#21370);
#19354=AXIS2_PLACEMENT_3D('',#26608,#21371,#21372);
#19355=AXIS2_PLACEMENT_3D('',#26611,#21374,#21375);
#19356=AXIS2_PLACEMENT_3D('',#26612,#21376,#21377);
#19357=AXIS2_PLACEMENT_3D('',#26618,#21381,#21382);
#19358=AXIS2_PLACEMENT_3D('',#26624,#21386,#21387);
#19359=AXIS2_PLACEMENT_3D('',#26627,#21390,#21391);
#19360=AXIS2_PLACEMENT_3D('',#26628,#21392,#21393);
#21200=DIRECTION('axis',(0.,0.,1.));
#21201=DIRECTION('refdir',(1.,0.,0.));
#21202=DIRECTION('center_axis',(0.,0.,1.));
#21203=DIRECTION('ref_axis',(1.,0.,0.));
#21204=DIRECTION('center_axis',(0.,0.,1.));
#21205=DIRECTION('ref_axis',(1.,0.,0.));
#21206=DIRECTION('',(0.,0.,1.));
#21207=DIRECTION('center_axis',(0.,0.,-1.));
#21208=DIRECTION('ref_axis',(1.,0.,0.));
#21209=DIRECTION('center_axis',(0.,1.,0.));
#21210=DIRECTION('ref_axis',(0.,0.,1.));
#21211=DIRECTION('',(0.,0.,-1.));
#21212=DIRECTION('',(1.,0.,0.));
#21213=DIRECTION('',(0.,0.,-1.));
#21214=DIRECTION('',(-1.,0.,0.));
#21215=DIRECTION('center_axis',(1.,0.,0.));
#21216=DIRECTION('ref_axis',(0.,0.,-1.));
#21217=DIRECTION('',(0.,0.,1.));
#21218=DIRECTION('',(0.,1.,0.));
#21219=DIRECTION('',(0.,1.,0.));
#21220=DIRECTION('center_axis',(0.,1.,0.));
#21221=DIRECTION('ref_axis',(1.,0.,0.));
#21222=DIRECTION('',(0.,0.,1.));
#21223=DIRECTION('',(1.,0.,0.));
#21224=DIRECTION('',(-1.,0.,0.));
#21225=DIRECTION('center_axis',(1.,0.,0.));
#21226=DIRECTION('ref_axis',(0.,1.,0.));
#21227=DIRECTION('',(0.,1.,0.));
#21228=DIRECTION('',(0.,0.,1.));
#21229=DIRECTION('',(0.,1.,0.));
#21230=DIRECTION('center_axis',(1.,0.,0.));
#21231=DIRECTION('ref_axis',(0.,1.,0.));
#21232=DIRECTION('',(0.,1.,0.));
#21233=DIRECTION('',(0.,0.,1.));
#21234=DIRECTION('',(0.,1.,0.));
#21235=DIRECTION('center_axis',(0.,0.,1.));
#21236=DIRECTION('ref_axis',(1.,0.,0.));
#21237=DIRECTION('center_axis',(0.,0.,1.));
#21238=DIRECTION('ref_axis',(1.,0.,0.));
#21239=DIRECTION('',(0.,0.,1.));
#21240=DIRECTION('center_axis',(0.,0.,-1.));
#21241=DIRECTION('ref_axis',(1.,0.,0.));
#21242=DIRECTION('center_axis',(0.,0.,1.));
#21243=DIRECTION('ref_axis',(1.,0.,0.));
#21244=DIRECTION('center_axis',(0.,0.,1.));
#21245=DIRECTION('ref_axis',(1.,0.,0.));
#21246=DIRECTION('center_axis',(0.,0.,1.));
#21247=DIRECTION('ref_axis',(1.,0.,0.));
#21248=DIRECTION('',(0.,0.,1.));
#21249=DIRECTION('center_axis',(0.,0.,-1.));
#21250=DIRECTION('ref_axis',(1.,0.,0.));
#21251=DIRECTION('center_axis',(0.,0.,1.));
#21252=DIRECTION('ref_axis',(1.,0.,0.));
#21253=DIRECTION('center_axis',(0.,0.,1.));
#21254=DIRECTION('ref_axis',(1.,0.,0.));
#21255=DIRECTION('center_axis',(0.,0.,1.));
#21256=DIRECTION('ref_axis',(1.,0.,0.));
#21257=DIRECTION('',(0.,0.,1.));
#21258=DIRECTION('center_axis',(0.,0.,-1.));
#21259=DIRECTION('ref_axis',(1.,0.,0.));
#21260=DIRECTION('center_axis',(0.,0.,1.));
#21261=DIRECTION('ref_axis',(1.,0.,0.));
#21262=DIRECTION('center_axis',(0.,0.,1.));
#21263=DIRECTION('ref_axis',(1.,0.,0.));
#21264=DIRECTION('center_axis',(0.,0.,1.));
#21265=DIRECTION('ref_axis',(1.,0.,0.));
#21266=DIRECTION('',(0.,0.,1.));
#21267=DIRECTION('center_axis',(0.,0.,-1.));
#21268=DIRECTION('ref_axis',(1.,0.,0.));
#21269=DIRECTION('center_axis',(0.,0.,1.));
#21270=DIRECTION('ref_axis',(1.,0.,0.));
#21271=DIRECTION('center_axis',(0.,0.,1.));
#21272=DIRECTION('ref_axis',(1.,0.,0.));
#21273=DIRECTION('center_axis',(0.,0.,1.));
#21274=DIRECTION('ref_axis',(1.,0.,0.));
#21275=DIRECTION('',(0.,0.,1.));
#21276=DIRECTION('center_axis',(0.,0.,-1.));
#21277=DIRECTION('ref_axis',(1.,0.,0.));
#21278=DIRECTION('center_axis',(0.,0.,1.));
#21279=DIRECTION('ref_axis',(1.,0.,0.));
#21280=DIRECTION('center_axis',(0.,0.,1.));
#21281=DIRECTION('ref_axis',(1.,0.,0.));
#21282=DIRECTION('',(0.,0.,1.));
#21283=DIRECTION('center_axis',(0.,0.,-1.));
#21284=DIRECTION('ref_axis',(1.,0.,0.));
#21285=DIRECTION('center_axis',(0.,0.,1.));
#21286=DIRECTION('ref_axis',(1.,0.,0.));
#21287=DIRECTION('center_axis',(0.,0.,1.));
#21288=DIRECTION('ref_axis',(1.,0.,0.));
#21289=DIRECTION('',(0.,0.,1.));
#21290=DIRECTION('center_axis',(0.,0.,-1.));
#21291=DIRECTION('ref_axis',(1.,0.,0.));
#21292=DIRECTION('center_axis',(0.,0.,1.));
#21293=DIRECTION('ref_axis',(1.,0.,0.));
#21294=DIRECTION('center_axis',(0.,0.,1.));
#21295=DIRECTION('ref_axis',(1.,0.,0.));
#21296=DIRECTION('',(0.,0.,1.));
#21297=DIRECTION('center_axis',(0.,0.,-1.));
#21298=DIRECTION('ref_axis',(1.,0.,0.));
#21299=DIRECTION('center_axis',(0.,0.,1.));
#21300=DIRECTION('ref_axis',(1.,0.,0.));
#21301=DIRECTION('center_axis',(0.,0.,1.));
#21302=DIRECTION('ref_axis',(1.,0.,0.));
#21303=DIRECTION('',(0.,0.,1.));
#21304=DIRECTION('center_axis',(0.,0.,-1.));
#21305=DIRECTION('ref_axis',(1.,0.,0.));
#21306=DIRECTION('center_axis',(0.,0.,1.));
#21307=DIRECTION('ref_axis',(1.,0.,0.));
#21308=DIRECTION('center_axis',(0.,0.,1.));
#21309=DIRECTION('ref_axis',(1.,0.,0.));
#21310=DIRECTION('',(0.,0.,1.));
#21311=DIRECTION('center_axis',(0.,0.,-1.));
#21312=DIRECTION('ref_axis',(1.,0.,0.));
#21313=DIRECTION('center_axis',(0.,0.,1.));
#21314=DIRECTION('ref_axis',(1.,0.,0.));
#21315=DIRECTION('center_axis',(0.,0.,1.));
#21316=DIRECTION('ref_axis',(1.,0.,0.));
#21317=DIRECTION('',(0.,0.,1.));
#21318=DIRECTION('center_axis',(0.,0.,-1.));
#21319=DIRECTION('ref_axis',(1.,0.,0.));
#21320=DIRECTION('center_axis',(0.,0.,1.));
#21321=DIRECTION('ref_axis',(1.,0.,0.));
#21322=DIRECTION('center_axis',(0.,0.,1.));
#21323=DIRECTION('ref_axis',(1.,0.,0.));
#21324=DIRECTION('',(0.,0.,1.));
#21325=DIRECTION('center_axis',(0.,0.,-1.));
#21326=DIRECTION('ref_axis',(1.,0.,0.));
#21327=DIRECTION('center_axis',(0.,0.,1.));
#21328=DIRECTION('ref_axis',(1.,0.,0.));
#21329=DIRECTION('center_axis',(0.,0.,1.));
#21330=DIRECTION('ref_axis',(1.,0.,0.));
#21331=DIRECTION('',(0.,0.,1.));
#21332=DIRECTION('center_axis',(0.,0.,-1.));
#21333=DIRECTION('ref_axis',(1.,0.,0.));
#21334=DIRECTION('center_axis',(0.,0.,1.));
#21335=DIRECTION('ref_axis',(1.,0.,0.));
#21336=DIRECTION('center_axis',(0.,0.,1.));
#21337=DIRECTION('ref_axis',(1.,0.,0.));
#21338=DIRECTION('',(0.,0.,1.));
#21339=DIRECTION('center_axis',(0.,0.,-1.));
#21340=DIRECTION('ref_axis',(1.,0.,0.));
#21341=DIRECTION('center_axis',(0.,0.,1.));
#21342=DIRECTION('ref_axis',(1.,0.,0.));
#21343=DIRECTION('center_axis',(0.,0.,1.));
#21344=DIRECTION('ref_axis',(1.,0.,0.));
#21345=DIRECTION('',(0.,0.,1.));
#21346=DIRECTION('center_axis',(0.,0.,-1.));
#21347=DIRECTION('ref_axis',(1.,0.,0.));
#21348=DIRECTION('center_axis',(0.,0.,1.));
#21349=DIRECTION('ref_axis',(1.,0.,0.));
#21350=DIRECTION('center_axis',(0.,0.,1.));
#21351=DIRECTION('ref_axis',(1.,0.,0.));
#21352=DIRECTION('',(0.,0.,1.));
#21353=DIRECTION('center_axis',(0.,0.,-1.));
#21354=DIRECTION('ref_axis',(1.,0.,0.));
#21355=DIRECTION('center_axis',(0.,0.,1.));
#21356=DIRECTION('ref_axis',(1.,0.,0.));
#21357=DIRECTION('center_axis',(0.,0.,1.));
#21358=DIRECTION('ref_axis',(1.,0.,0.));
#21359=DIRECTION('',(0.,0.,1.));
#21360=DIRECTION('center_axis',(0.,0.,-1.));
#21361=DIRECTION('ref_axis',(1.,0.,0.));
#21362=DIRECTION('center_axis',(0.,0.,1.));
#21363=DIRECTION('ref_axis',(1.,0.,0.));
#21364=DIRECTION('center_axis',(0.,0.,1.));
#21365=DIRECTION('ref_axis',(1.,0.,0.));
#21366=DIRECTION('',(0.,0.,1.));
#21367=DIRECTION('center_axis',(0.,0.,-1.));
#21368=DIRECTION('ref_axis',(1.,0.,0.));
#21369=DIRECTION('center_axis',(0.,0.,1.));
#21370=DIRECTION('ref_axis',(1.,0.,0.));
#21371=DIRECTION('center_axis',(0.,0.,1.));
#21372=DIRECTION('ref_axis',(1.,0.,0.));
#21373=DIRECTION('',(0.,0.,1.));
#21374=DIRECTION('center_axis',(0.,0.,-1.));
#21375=DIRECTION('ref_axis',(1.,0.,0.));
#21376=DIRECTION('center_axis',(0.,1.,0.));
#21377=DIRECTION('ref_axis',(-1.,0.,0.));
#21378=DIRECTION('',(-1.,0.,0.));
#21379=DIRECTION('',(0.,0.,1.));
#21380=DIRECTION('',(-1.,0.,0.));
#21381=DIRECTION('center_axis',(0.,-1.,0.));
#21382=DIRECTION('ref_axis',(1.,0.,0.));
#21383=DIRECTION('',(1.,0.,0.));
#21384=DIRECTION('',(1.,0.,0.));
#21385=DIRECTION('',(0.,0.,1.));
#21386=DIRECTION('center_axis',(-1.,0.,0.));
#21387=DIRECTION('ref_axis',(0.,-1.,0.));
#21388=DIRECTION('',(0.,-1.,0.));
#21389=DIRECTION('',(0.,-1.,0.));
#21390=DIRECTION('center_axis',(0.,0.,1.));
#21391=DIRECTION('ref_axis',(1.,0.,0.));
#21392=DIRECTION('center_axis',(0.,0.,1.));
#21393=DIRECTION('ref_axis',(1.,0.,0.));
#26454=CARTESIAN_POINT('',(0.,0.,0.));
#26455=CARTESIAN_POINT('Origin',(10.,0.,-1.3));
#26456=CARTESIAN_POINT('',(9.725,-3.36777869765523E-17,-1.2));
#26457=CARTESIAN_POINT('Origin',(10.,0.,-1.2));
#26458=CARTESIAN_POINT('',(9.725,3.36777869765523E-17,0.));
#26459=CARTESIAN_POINT('',(9.725,-3.36777869765523E-17,-1.3));
#26460=CARTESIAN_POINT('Origin',(10.,0.,0.));
#26461=CARTESIAN_POINT('Origin',(10.,2.,-0.6));
#26462=CARTESIAN_POINT('',(9.,2.,0.));
#26463=CARTESIAN_POINT('',(9.,2.,-1.2));
#26464=CARTESIAN_POINT('',(9.,2.,-0.9));
#26465=CARTESIAN_POINT('',(12.,2.,0.));
#26466=CARTESIAN_POINT('',(12.,2.,0.));
#26467=CARTESIAN_POINT('',(12.,2.,-1.2));
#26468=CARTESIAN_POINT('',(12.,2.,-1.2));
#26469=CARTESIAN_POINT('',(8.,2.,-1.2));
#26470=CARTESIAN_POINT('Origin',(12.,-2.,0.));
#26471=CARTESIAN_POINT('',(12.,-2.,-1.2));
#26472=CARTESIAN_POINT('',(12.,-2.,0.));
#26473=CARTESIAN_POINT('',(12.,-2.,-1.2));
#26474=CARTESIAN_POINT('',(12.,-2.,-1.2));
#26475=CARTESIAN_POINT('',(12.,-2.,0.));
#26476=CARTESIAN_POINT('Origin',(10.,-2.,-0.6));
#26477=CARTESIAN_POINT('',(9.,-2.,-1.2));
#26478=CARTESIAN_POINT('',(9.,-2.,0.));
#26479=CARTESIAN_POINT('',(9.,-2.,-0.9));
#26480=CARTESIAN_POINT('',(8.,-2.,-1.2));
#26481=CARTESIAN_POINT('',(12.,-2.,0.));
#26482=CARTESIAN_POINT('Origin',(9.,-4.5,-1.2));
#26483=CARTESIAN_POINT('',(9.,12.5,-1.2));
#26484=CARTESIAN_POINT('',(9.,-4.5,-1.2));
#26485=CARTESIAN_POINT('',(9.,12.5,0.));
#26486=CARTESIAN_POINT('',(9.,12.5,-1.2));
#26487=CARTESIAN_POINT('',(9.,-4.5,0.));
#26488=CARTESIAN_POINT('Origin',(9.,-4.5,-1.2));
#26489=CARTESIAN_POINT('',(9.,-4.5,0.));
#26490=CARTESIAN_POINT('',(9.,-4.5,0.));
#26491=CARTESIAN_POINT('',(9.,-4.5,-1.2));
#26492=CARTESIAN_POINT('',(9.,-4.5,-1.2));
#26493=CARTESIAN_POINT('',(9.,-4.5,-1.2));
#26494=CARTESIAN_POINT('Origin',(-2.5,-1.5,-1.1));
#26495=CARTESIAN_POINT('',(-2.665,-1.5,-1.1));
#26496=CARTESIAN_POINT('Origin',(-2.5,-1.5,-1.1));
#26497=CARTESIAN_POINT('',(-2.665,-1.5,0.));
#26498=CARTESIAN_POINT('',(-2.665,-1.5,-1.1));
#26499=CARTESIAN_POINT('Origin',(-2.5,-1.5,0.));
#26500=CARTESIAN_POINT('Origin',(-2.5,-1.5,-1.1));
#26501=CARTESIAN_POINT('Origin',(1.53080849893419E-16,1.,-1.1));
#26502=CARTESIAN_POINT('',(-0.165,1.,-1.1));
#26503=CARTESIAN_POINT('Origin',(1.53080849893419E-16,1.,-1.1));
#26504=CARTESIAN_POINT('',(-0.165,1.,0.));
#26505=CARTESIAN_POINT('',(-0.165,1.,-1.1));
#26506=CARTESIAN_POINT('Origin',(1.53080849893419E-16,1.,0.));
#26507=CARTESIAN_POINT('Origin',(1.66533453693773E-16,1.,-1.1));
#26508=CARTESIAN_POINT('Origin',(2.5,-1.5,-1.1));
#26509=CARTESIAN_POINT('',(2.335,-1.5,-1.1));
#26510=CARTESIAN_POINT('Origin',(2.5,-1.5,-1.1));
#26511=CARTESIAN_POINT('',(2.335,-1.5,0.));
#26512=CARTESIAN_POINT('',(2.335,-1.5,-1.1));
#26513=CARTESIAN_POINT('Origin',(2.5,-1.5,0.));
#26514=CARTESIAN_POINT('Origin',(2.5,-1.5,-1.1));
#26515=CARTESIAN_POINT('Origin',(-4.59242549680257E-16,-4.,-1.1));
#26516=CARTESIAN_POINT('',(-0.165,-4.,-1.1));
#26517=CARTESIAN_POINT('Origin',(-4.59242549680257E-16,-4.,-1.1));
#26518=CARTESIAN_POINT('',(-0.165,-4.,0.));
#26519=CARTESIAN_POINT('',(-0.165,-4.,-1.1));
#26520=CARTESIAN_POINT('Origin',(-4.59242549680257E-16,-4.,0.));
#26521=CARTESIAN_POINT('Origin',(-4.71844785465692E-16,-4.,-1.1));
#26522=CARTESIAN_POINT('Origin',(6.,5.,-1.3));
#26523=CARTESIAN_POINT('',(5.725,5.,-1.2));
#26524=CARTESIAN_POINT('Origin',(6.,5.,-1.2));
#26525=CARTESIAN_POINT('',(5.725,5.,0.));
#26526=CARTESIAN_POINT('',(5.725,5.,-1.3));
#26527=CARTESIAN_POINT('Origin',(6.,5.,0.));
#26528=CARTESIAN_POINT('Origin',(-6.,5.,-1.3));
#26529=CARTESIAN_POINT('',(-6.275,5.,-1.2));
#26530=CARTESIAN_POINT('Origin',(-6.,5.,-1.2));
#26531=CARTESIAN_POINT('',(-6.275,5.,0.));
#26532=CARTESIAN_POINT('',(-6.275,5.,-1.3));
#26533=CARTESIAN_POINT('Origin',(-6.,5.,0.));
#26534=CARTESIAN_POINT('Origin',(2.5,2.5,-1.3));
#26535=CARTESIAN_POINT('',(2.225,2.5,-1.2));
#26536=CARTESIAN_POINT('Origin',(2.5,2.5,-1.2));
#26537=CARTESIAN_POINT('',(2.225,2.5,0.));
#26538=CARTESIAN_POINT('',(2.225,2.5,-1.3));
#26539=CARTESIAN_POINT('Origin',(2.5,2.5,0.));
#26540=CARTESIAN_POINT('Origin',(-2.5,7.5,-1.3));
#26541=CARTESIAN_POINT('',(-2.775,7.5,-1.2));
#26542=CARTESIAN_POINT('Origin',(-2.5,7.5,-1.2));
#26543=CARTESIAN_POINT('',(-2.775,7.5,0.));
#26544=CARTESIAN_POINT('',(-2.775,7.5,-1.3));
#26545=CARTESIAN_POINT('Origin',(-2.5,7.5,0.));
#26546=CARTESIAN_POINT('Origin',(-2.5,2.5,-1.3));
#26547=CARTESIAN_POINT('',(-2.775,2.5,-1.2));
#26548=CARTESIAN_POINT('Origin',(-2.5,2.5,-1.2));
#26549=CARTESIAN_POINT('',(-2.775,2.5,0.));
#26550=CARTESIAN_POINT('',(-2.775,2.5,-1.3));
#26551=CARTESIAN_POINT('Origin',(-2.5,2.5,0.));
#26552=CARTESIAN_POINT('Origin',(2.5,7.5,-1.3));
#26553=CARTESIAN_POINT('',(2.225,7.5,-1.2));
#26554=CARTESIAN_POINT('Origin',(2.5,7.5,-1.2));
#26555=CARTESIAN_POINT('',(2.225,7.5,0.));
#26556=CARTESIAN_POINT('',(2.225,7.5,-1.3));
#26557=CARTESIAN_POINT('Origin',(2.5,7.5,0.));
#26558=CARTESIAN_POINT('Origin',(0.,5.,-1.3));
#26559=CARTESIAN_POINT('',(-2.5,5.,-1.2));
#26560=CARTESIAN_POINT('Origin',(0.,5.,-1.2));
#26561=CARTESIAN_POINT('',(-2.5,5.,0.));
#26562=CARTESIAN_POINT('',(-2.5,5.,-1.3));
#26563=CARTESIAN_POINT('Origin',(0.,5.,0.));
#26564=CARTESIAN_POINT('Origin',(4.4,2.7,-1.3));
#26565=CARTESIAN_POINT('',(4.125,2.7,-1.2));
#26566=CARTESIAN_POINT('Origin',(4.4,2.7,-1.2));
#26567=CARTESIAN_POINT('',(4.125,2.7,0.));
#26568=CARTESIAN_POINT('',(4.125,2.7,-1.3));
#26569=CARTESIAN_POINT('Origin',(4.4,2.7,0.));
#26570=CARTESIAN_POINT('Origin',(7.6,2.7,-1.3));
#26571=CARTESIAN_POINT('',(7.325,2.7,-1.2));
#26572=CARTESIAN_POINT('Origin',(7.6,2.7,-1.2));
#26573=CARTESIAN_POINT('',(7.325,2.7,0.));
#26574=CARTESIAN_POINT('',(7.325,2.7,-1.3));
#26575=CARTESIAN_POINT('Origin',(7.6,2.7,0.));
#26576=CARTESIAN_POINT('Origin',(-7.6,2.7,-1.3));
#26577=CARTESIAN_POINT('',(-7.875,2.7,-1.2));
#26578=CARTESIAN_POINT('Origin',(-7.6,2.7,-1.2));
#26579=CARTESIAN_POINT('',(-7.875,2.7,0.));
#26580=CARTESIAN_POINT('',(-7.875,2.7,-1.3));
#26581=CARTESIAN_POINT('Origin',(-7.6,2.7,0.));
#26582=CARTESIAN_POINT('Origin',(-4.4,2.7,-1.3));
#26583=CARTESIAN_POINT('',(-4.675,2.7,-1.2));
#26584=CARTESIAN_POINT('Origin',(-4.4,2.7,-1.2));
#26585=CARTESIAN_POINT('',(-4.675,2.7,0.));
#26586=CARTESIAN_POINT('',(-4.675,2.7,-1.3));
#26587=CARTESIAN_POINT('Origin',(-4.4,2.7,0.));
#26588=CARTESIAN_POINT('Origin',(7.,9.5,-1.3));
#26589=CARTESIAN_POINT('',(6.725,9.5,-1.2));
#26590=CARTESIAN_POINT('Origin',(7.,9.5,-1.2));
#26591=CARTESIAN_POINT('',(6.725,9.5,0.));
#26592=CARTESIAN_POINT('',(6.725,9.5,-1.3));
#26593=CARTESIAN_POINT('Origin',(7.,9.5,0.));
#26594=CARTESIAN_POINT('Origin',(7.,10.5,-1.3));
#26595=CARTESIAN_POINT('',(6.725,10.5,-1.2));
#26596=CARTESIAN_POINT('Origin',(7.,10.5,-1.2));
#26597=CARTESIAN_POINT('',(6.725,10.5,0.));
#26598=CARTESIAN_POINT('',(6.725,10.5,-1.3));
#26599=CARTESIAN_POINT('Origin',(7.,10.5,0.));
#26600=CARTESIAN_POINT('Origin',(-7.,9.5,-1.3));
#26601=CARTESIAN_POINT('',(-7.275,9.5,-1.2));
#26602=CARTESIAN_POINT('Origin',(-7.,9.5,-1.2));
#26603=CARTESIAN_POINT('',(-7.275,9.5,0.));
#26604=CARTESIAN_POINT('',(-7.275,9.5,-1.3));
#26605=CARTESIAN_POINT('Origin',(-7.,9.5,0.));
#26606=CARTESIAN_POINT('Origin',(-7.,10.5,-1.3));
#26607=CARTESIAN_POINT('',(-7.275,10.5,-1.2));
#26608=CARTESIAN_POINT('Origin',(-7.,10.5,-1.2));
#26609=CARTESIAN_POINT('',(-7.275,10.5,0.));
#26610=CARTESIAN_POINT('',(-7.275,10.5,-1.3));
#26611=CARTESIAN_POINT('Origin',(-7.,10.5,0.));
#26612=CARTESIAN_POINT('Origin',(9.,12.5,-1.2));
#26613=CARTESIAN_POINT('',(-9.,12.5,-1.2));
#26614=CARTESIAN_POINT('',(9.,12.5,-1.2));
#26615=CARTESIAN_POINT('',(-9.,12.5,0.));
#26616=CARTESIAN_POINT('',(-9.,12.5,-1.2));
#26617=CARTESIAN_POINT('',(9.,12.5,0.));
#26618=CARTESIAN_POINT('Origin',(-9.,-4.5,-1.2));
#26619=CARTESIAN_POINT('',(-9.,-4.5,-1.2));
#26620=CARTESIAN_POINT('',(-9.,-4.5,-1.2));
#26621=CARTESIAN_POINT('',(-9.,-4.5,0.));
#26622=CARTESIAN_POINT('',(-9.,-4.5,0.));
#26623=CARTESIAN_POINT('',(-9.,-4.5,-1.2));
#26624=CARTESIAN_POINT('Origin',(-9.,12.5,-1.2));
#26625=CARTESIAN_POINT('',(-9.,12.5,-1.2));
#26626=CARTESIAN_POINT('',(-9.,12.5,0.));
#26627=CARTESIAN_POINT('Origin',(0.,4.,0.));
#26628=CARTESIAN_POINT('Origin',(0.,4.,-1.2));
#43388=UNCERTAINTY_MEASURE_WITH_UNIT(LENGTH_MEASURE(0.001),#43522,
'DISTANCE_ACCURACY_VALUE',
'Maximum model space distance between geometric entities at asserted c
onnectivities');
#43453=UNCERTAINTY_MEASURE_WITH_UNIT(LENGTH_MEASURE(0.001),#43522,
'DISTANCE_ACCURACY_VALUE',
'Maximum model space distance between geometric entities at asserted c
onnectivities');
#43456=(
GEOMETRIC_REPRESENTATION_CONTEXT(3)
GLOBAL_UNCERTAINTY_ASSIGNED_CONTEXT((#43388))
GLOBAL_UNIT_ASSIGNED_CONTEXT((#43522,#43524,#43525))
REPRESENTATION_CONTEXT('','3D')
);
#43521=(
GEOMETRIC_REPRESENTATION_CONTEXT(3)
GLOBAL_UNCERTAINTY_ASSIGNED_CONTEXT((#43453))
GLOBAL_UNIT_ASSIGNED_CONTEXT((#43522,#43524,#43525))
REPRESENTATION_CONTEXT('','3D')
);
#43522=(
LENGTH_UNIT()
NAMED_UNIT(*)
SI_UNIT(.CENTI.,.METRE.)
);
#43524=(
NAMED_UNIT(*)
PLANE_ANGLE_UNIT()
SI_UNIT($,.RADIAN.)
);
#43525=(
NAMED_UNIT(*)
SI_UNIT($,.STERADIAN.)
SOLID_ANGLE_UNIT()
);
#43528=SHAPE_DEFINITION_REPRESENTATION(#43595,#43796);
#43595=PRODUCT_DEFINITION_SHAPE('',$,#43864);
#43796=SHAPE_REPRESENTATION('',(#19286),#43456);
#43861=PRODUCT_DEFINITION_CONTEXT('part definition',#44064,'design');
#43864=PRODUCT_DEFINITION('Base','Base',#43931,#43861);
#43931=PRODUCT_DEFINITION_FORMATION('',$,#44068);
#44064=APPLICATION_CONTEXT(
'Core Data for Automotive Mechanical Design Process');
#44065=PRODUCT_CONTEXT('part definition',#44064,'mechanical');
#44068=PRODUCT('Base','Base','Base',(#44065));
#44175=COLOUR_RGB('Dark Blue',0.08,0.2,0.34);
#44176=FILL_AREA_STYLE_COLOUR('',#44175);
#44177=FILL_AREA_STYLE('',(#44176));
#44178=SURFACE_STYLE_FILL_AREA(#44177);
#44179=SURFACE_SIDE_STYLE('',(#44178));
#44180=SURFACE_STYLE_USAGE(.BOTH.,#44179);
#44181=PRESENTATION_STYLE_ASSIGNMENT((#44180));
ENDSEC;
END-ISO-10303-21;
